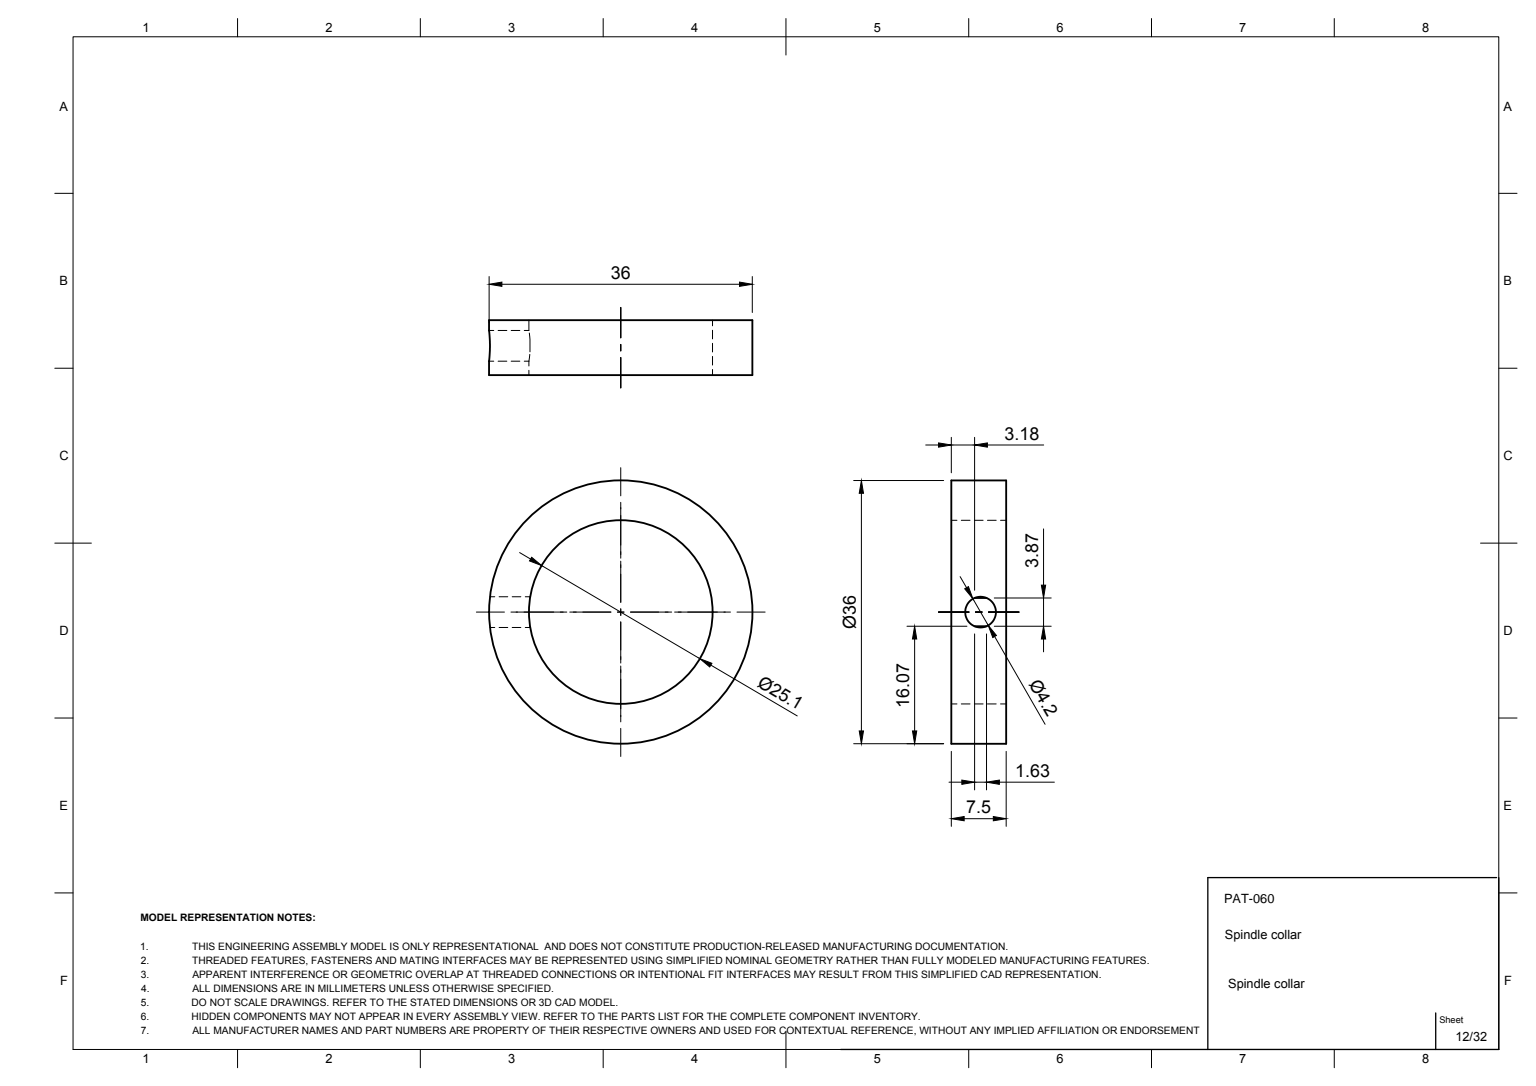
ISO-10303-21;
HEADER;
/* Generated by software containing ST-Developer
 * from STEP Tools, Inc. (www.steptools.com) 
 */

FILE_DESCRIPTION(
/* description */ ('Indexing fixture plate with plunger'),
/* implementation_level */ '2;1');

FILE_NAME(
/* name */ 'Spindle collar.step',
/* time_stamp */ '2026-10-28T03:23:41-07:00',
/* author */ (''),
/* organization */ (''),
/* preprocessor_version */ 'ST-DEVELOPER v20.2',
/* originating_system */ 'Autodesk Translation Framework v15.17.0.0',
/* authorisation */ '');

FILE_SCHEMA (('AUTOMOTIVE_DESIGN { 1 0 10303 214 3 1 1 }'));
ENDSEC;

DATA;
#10=MECHANICAL_DESIGN_GEOMETRIC_PRESENTATION_REPRESENTATION('',(#324),#10020);
#234=B_SPLINE_CURVE_WITH_KNOTS('',3,(#7309,#7310,#7311,#7312,#7313,#7314,
#7315,#7316,#7317,#7318,#7319,#7320,#7321,#7322),.UNSPECIFIED.,.F.,.F.,
(4,2,2,2,2,2,4),(0.714680326757343,0.792648662700719,0.871912238073926,
0.951175813447133,1.03043938882034,1.10970296419355,1.18767130013692),
 .UNSPECIFIED.);
#235=B_SPLINE_CURVE_WITH_KNOTS('',3,(#7326,#7327,#7328,#7329,#7330,#7331,
#7332,#7333),.UNSPECIFIED.,.F.,.F.,(4,2,2,4),(0.317058604482378,0.396322179855585,
0.475585755228792,0.55355409117217),.UNSPECIFIED.);
#236=B_SPLINE_CURVE_WITH_KNOTS('',3,(#7337,#7338,#7339,#7340,#7341,#7342,
#7343,#7344,#7345,#7346,#7347,#7348,#7349,#7350,#7351,#7352,#7353,#7354,
#7355,#7356,#7357,#7358,#7359,#7360,#7361,#7362),.UNSPECIFIED.,.F.,.F.,
(4,2,2,2,2,2,2,2,2,2,2,2,4),(0.,0.0791819055472369,0.158363811094474,0.237545215630596,
0.316726620166718,0.395908024702839,0.475089429238961,0.554271334786198,
0.633453240333435,0.712635145880672,0.791817051427909,0.870998455964031,
0.950179860500153),.UNSPECIFIED.);
#237=B_SPLINE_CURVE_WITH_KNOTS('',3,(#7363,#7364,#7365,#7366,#7367,#7368,
#7369,#7370,#7371,#7372),.UNSPECIFIED.,.F.,.F.,(4,2,2,2,4),(0.950179860500153,
1.02936126503627,1.1085426695724,1.18772457511963,1.26690648066687),
 .UNSPECIFIED.);
#238=B_SPLINE_CURVE_WITH_KNOTS('',3,(#7373,#7374,#7375,#7376,#7377,#7378,
#7379,#7380),.UNSPECIFIED.,.F.,.F.,(4,2,2,4),(0.0805631177925868,0.158531453735964,
0.237795029109171,0.317058604482378),.UNSPECIFIED.);
#270=SHAPE_REPRESENTATION_RELATIONSHIP('SRR','None',#10144,#297);
#297=ADVANCED_BREP_SHAPE_REPRESENTATION('',(#360),#9997);
#324=STYLED_ITEM('',(#10361),#360);
#360=MANIFOLD_SOLID_BREP('Body1',#4578);
#414=FACE_BOUND('',#1029,.T.);
#415=FACE_BOUND('',#1031,.T.);
#416=FACE_BOUND('',#1033,.T.);
#417=FACE_BOUND('',#1035,.T.);
#558=PLANE('',#5001);
#559=PLANE('',#5005);
#560=PLANE('',#5012);
#561=PLANE('',#5013);
#712=FACE_OUTER_BOUND('',#1025,.T.);
#713=FACE_OUTER_BOUND('',#1026,.T.);
#714=FACE_OUTER_BOUND('',#1027,.T.);
#715=FACE_OUTER_BOUND('',#1028,.T.);
#716=FACE_OUTER_BOUND('',#1030,.T.);
#717=FACE_OUTER_BOUND('',#1032,.T.);
#718=FACE_OUTER_BOUND('',#1034,.T.);
#1025=EDGE_LOOP('',(#3213,#3214));
#1026=EDGE_LOOP('',(#3215,#3216,#3217,#3218,#3219,#3220,#3221,#3222,#3223));
#1027=EDGE_LOOP('',(#3224,#3225));
#1028=EDGE_LOOP('',(#3226,#3227,#3228,#3229));
#1029=EDGE_LOOP('',(#3230,#3231,#3232,#3233,#3234));
#1030=EDGE_LOOP('',(#3235,#3236,#3237,#3238));
#1031=EDGE_LOOP('',(#3239,#3240));
#1032=EDGE_LOOP('',(#3241));
#1033=EDGE_LOOP('',(#3242));
#1034=EDGE_LOOP('',(#3243));
#1035=EDGE_LOOP('',(#3244));
#1425=LINE('',#7305,#1645);
#1426=LINE('',#7335,#1646);
#1427=LINE('',#7382,#1647);
#1428=LINE('',#7387,#1648);
#1429=LINE('',#7393,#1649);
#1645=VECTOR('',#5796,1.);
#1646=VECTOR('',#5803,0.21);
#1647=VECTOR('',#5806,1.);
#1648=VECTOR('',#5811,1.255);
#1649=VECTOR('',#5818,1.8);
#1874=CIRCLE('',#5002,0.21);
#1875=CIRCLE('',#5004,0.21);
#1876=CIRCLE('',#5007,1.255);
#1877=CIRCLE('',#5008,1.255);
#1878=CIRCLE('',#5010,1.8);
#1879=CIRCLE('',#5011,1.8);
#2185=VERTEX_POINT('',#7303);
#2186=VERTEX_POINT('',#7304);
#2187=VERTEX_POINT('',#7308);
#2188=VERTEX_POINT('',#7323);
#2189=VERTEX_POINT('',#7325);
#2190=VERTEX_POINT('',#7334);
#2191=VERTEX_POINT('',#7336);
#2192=VERTEX_POINT('',#7384);
#2193=VERTEX_POINT('',#7386);
#2194=VERTEX_POINT('',#7390);
#2195=VERTEX_POINT('',#7392);
#2586=EDGE_CURVE('',#2185,#2186,#1425,.T.);
#2587=EDGE_CURVE('',#2185,#2186,#1874,.T.);
#2588=EDGE_CURVE('',#2187,#2185,#234,.T.);
#2589=EDGE_CURVE('',#2188,#2187,#1875,.T.);
#2590=EDGE_CURVE('',#2189,#2188,#235,.T.);
#2591=EDGE_CURVE('',#2189,#2190,#1426,.T.);
#2592=EDGE_CURVE('',#2191,#2190,#236,.T.);
#2593=EDGE_CURVE('',#2190,#2191,#237,.T.);
#2594=EDGE_CURVE('',#2186,#2189,#238,.T.);
#2595=EDGE_CURVE('',#2188,#2187,#1427,.T.);
#2596=EDGE_CURVE('',#2192,#2192,#1876,.T.);
#2597=EDGE_CURVE('',#2192,#2193,#1428,.T.);
#2598=EDGE_CURVE('',#2193,#2193,#1877,.T.);
#2599=EDGE_CURVE('',#2194,#2194,#1878,.T.);
#2600=EDGE_CURVE('',#2194,#2195,#1429,.T.);
#2601=EDGE_CURVE('',#2195,#2195,#1879,.T.);
#3213=ORIENTED_EDGE('',*,*,#2586,.F.);
#3214=ORIENTED_EDGE('',*,*,#2587,.T.);
#3215=ORIENTED_EDGE('',*,*,#2588,.F.);
#3216=ORIENTED_EDGE('',*,*,#2589,.F.);
#3217=ORIENTED_EDGE('',*,*,#2590,.F.);
#3218=ORIENTED_EDGE('',*,*,#2591,.T.);
#3219=ORIENTED_EDGE('',*,*,#2592,.F.);
#3220=ORIENTED_EDGE('',*,*,#2593,.F.);
#3221=ORIENTED_EDGE('',*,*,#2591,.F.);
#3222=ORIENTED_EDGE('',*,*,#2594,.F.);
#3223=ORIENTED_EDGE('',*,*,#2587,.F.);
#3224=ORIENTED_EDGE('',*,*,#2595,.F.);
#3225=ORIENTED_EDGE('',*,*,#2589,.T.);
#3226=ORIENTED_EDGE('',*,*,#2596,.F.);
#3227=ORIENTED_EDGE('',*,*,#2597,.T.);
#3228=ORIENTED_EDGE('',*,*,#2598,.T.);
#3229=ORIENTED_EDGE('',*,*,#2597,.F.);
#3230=ORIENTED_EDGE('',*,*,#2594,.T.);
#3231=ORIENTED_EDGE('',*,*,#2590,.T.);
#3232=ORIENTED_EDGE('',*,*,#2595,.T.);
#3233=ORIENTED_EDGE('',*,*,#2588,.T.);
#3234=ORIENTED_EDGE('',*,*,#2586,.T.);
#3235=ORIENTED_EDGE('',*,*,#2599,.F.);
#3236=ORIENTED_EDGE('',*,*,#2600,.T.);
#3237=ORIENTED_EDGE('',*,*,#2601,.T.);
#3238=ORIENTED_EDGE('',*,*,#2600,.F.);
#3239=ORIENTED_EDGE('',*,*,#2592,.T.);
#3240=ORIENTED_EDGE('',*,*,#2593,.T.);
#3241=ORIENTED_EDGE('',*,*,#2599,.T.);
#3242=ORIENTED_EDGE('',*,*,#2596,.T.);
#3243=ORIENTED_EDGE('',*,*,#2601,.F.);
#3244=ORIENTED_EDGE('',*,*,#2598,.F.);
#4188=CYLINDRICAL_SURFACE('',#5003,0.21);
#4189=CYLINDRICAL_SURFACE('',#5006,1.255);
#4190=CYLINDRICAL_SURFACE('',#5009,1.8);
#4327=ADVANCED_FACE('',(#712),#558,.T.);
#4328=ADVANCED_FACE('',(#713),#4188,.F.);
#4329=ADVANCED_FACE('',(#714),#559,.T.);
#4330=ADVANCED_FACE('',(#715,#414),#4189,.F.);
#4331=ADVANCED_FACE('',(#716,#415),#4190,.T.);
#4332=ADVANCED_FACE('',(#717,#416),#560,.T.);
#4333=ADVANCED_FACE('',(#718,#417),#561,.F.);
#4578=CLOSED_SHELL('',(#4327,#4328,#4329,#4330,#4331,#4332,#4333));
#5000=AXIS2_PLACEMENT_3D('',#7301,#5792,#5793);
#5001=AXIS2_PLACEMENT_3D('',#7302,#5794,#5795);
#5002=AXIS2_PLACEMENT_3D('',#7306,#5797,#5798);
#5003=AXIS2_PLACEMENT_3D('',#7307,#5799,#5800);
#5004=AXIS2_PLACEMENT_3D('',#7324,#5801,#5802);
#5005=AXIS2_PLACEMENT_3D('',#7381,#5804,#5805);
#5006=AXIS2_PLACEMENT_3D('',#7383,#5807,#5808);
#5007=AXIS2_PLACEMENT_3D('',#7385,#5809,#5810);
#5008=AXIS2_PLACEMENT_3D('',#7388,#5812,#5813);
#5009=AXIS2_PLACEMENT_3D('',#7389,#5814,#5815);
#5010=AXIS2_PLACEMENT_3D('',#7391,#5816,#5817);
#5011=AXIS2_PLACEMENT_3D('',#7394,#5819,#5820);
#5012=AXIS2_PLACEMENT_3D('',#7395,#5821,#5822);
#5013=AXIS2_PLACEMENT_3D('',#7396,#5823,#5824);
#5792=DIRECTION('axis',(0.,0.,1.));
#5793=DIRECTION('refdir',(1.,0.,0.));
#5794=DIRECTION('center_axis',(1.,0.,0.));
#5795=DIRECTION('ref_axis',(0.,0.,-1.));
#5796=DIRECTION('',(0.,0.,1.));
#5797=DIRECTION('center_axis',(1.,0.,0.));
#5798=DIRECTION('ref_axis',(0.,0.,-1.));
#5799=DIRECTION('center_axis',(1.,0.,0.));
#5800=DIRECTION('ref_axis',(0.,0.,-1.));
#5801=DIRECTION('center_axis',(1.,0.,0.));
#5802=DIRECTION('ref_axis',(0.,0.,-1.));
#5803=DIRECTION('',(1.,0.,0.));
#5804=DIRECTION('center_axis',(1.,0.,0.));
#5805=DIRECTION('ref_axis',(0.,0.,-1.));
#5806=DIRECTION('',(0.,0.,-1.));
#5807=DIRECTION('center_axis',(0.,0.,1.));
#5808=DIRECTION('ref_axis',(1.,0.,0.));
#5809=DIRECTION('center_axis',(0.,0.,-1.));
#5810=DIRECTION('ref_axis',(1.,0.,0.));
#5811=DIRECTION('',(0.,0.,-1.));
#5812=DIRECTION('center_axis',(0.,0.,-1.));
#5813=DIRECTION('ref_axis',(1.,0.,0.));
#5814=DIRECTION('center_axis',(0.,0.,1.));
#5815=DIRECTION('ref_axis',(1.,0.,0.));
#5816=DIRECTION('center_axis',(0.,0.,1.));
#5817=DIRECTION('ref_axis',(1.,0.,0.));
#5818=DIRECTION('',(0.,0.,-1.));
#5819=DIRECTION('center_axis',(0.,0.,1.));
#5820=DIRECTION('ref_axis',(1.,0.,0.));
#5821=DIRECTION('center_axis',(0.,0.,1.));
#5822=DIRECTION('ref_axis',(1.,0.,0.));
#5823=DIRECTION('center_axis',(0.,0.,1.));
#5824=DIRECTION('ref_axis',(1.,0.,0.));
#7301=CARTESIAN_POINT('',(0.,0.,0.));
#7302=CARTESIAN_POINT('Origin',(1.24,0.,6.6));
#7303=CARTESIAN_POINT('',(1.24,0.19345542122153,6.51829932680816));
#7304=CARTESIAN_POINT('',(1.24,0.19345542122153,6.68170067319184));
#7305=CARTESIAN_POINT('',(1.24,0.193455421221531,6.25));
#7306=CARTESIAN_POINT('Origin',(1.24,0.,6.6));
#7307=CARTESIAN_POINT('Origin',(1.24,0.,6.6));
#7308=CARTESIAN_POINT('',(1.24,-0.19345542122153,6.51829932680816));
#7309=CARTESIAN_POINT('Ctrl Pts',(1.24,-0.193455421221531,6.51829932680816));
#7310=CARTESIAN_POINT('Ctrl Pts',(1.24167145707784,-0.182741806873435,6.49293103184137));
#7311=CARTESIAN_POINT('Ctrl Pts',(1.24400210952839,-0.16680484953796,6.46982000143961));
#7312=CARTESIAN_POINT('Ctrl Pts',(1.24840249136865,-0.129875785635207,6.43289093753686));
#7313=CARTESIAN_POINT('Ctrl Pts',(1.2507589672592,-0.106295060941802,6.4167372734261));
#7314=CARTESIAN_POINT('Ctrl Pts',(1.25408084670822,-0.0545698089447939,
6.39529044194989));
#7315=CARTESIAN_POINT('Ctrl Pts',(1.255,-0.0264211917910691,6.39));
#7316=CARTESIAN_POINT('Ctrl Pts',(1.255,0.026421191791069,6.39));
#7317=CARTESIAN_POINT('Ctrl Pts',(1.25408084670822,0.0545698089447938,6.39529044194989));
#7318=CARTESIAN_POINT('Ctrl Pts',(1.2507589672592,0.106295060941802,6.4167372734261));
#7319=CARTESIAN_POINT('Ctrl Pts',(1.24840249136865,0.129875785635207,6.43289093753686));
#7320=CARTESIAN_POINT('Ctrl Pts',(1.24400210952839,0.166804849537961,6.46982000143961));
#7321=CARTESIAN_POINT('Ctrl Pts',(1.24167145707784,0.182741806873435,6.49293103184137));
#7322=CARTESIAN_POINT('Ctrl Pts',(1.24,0.193455421221531,6.51829932680816));
#7323=CARTESIAN_POINT('',(1.24,-0.19345542122153,6.68170067319184));
#7324=CARTESIAN_POINT('Origin',(1.24,0.,6.6));
#7325=CARTESIAN_POINT('',(1.255,-5.44921548144906E-17,6.81));
#7326=CARTESIAN_POINT('Ctrl Pts',(1.255,-3.46944695195361E-17,6.81));
#7327=CARTESIAN_POINT('Ctrl Pts',(1.255,-0.0264211917910691,6.81));
#7328=CARTESIAN_POINT('Ctrl Pts',(1.25408084670822,-0.0545698089447938,
6.80470955805011));
#7329=CARTESIAN_POINT('Ctrl Pts',(1.2507589672592,-0.106295060941802,6.7832627265739));
#7330=CARTESIAN_POINT('Ctrl Pts',(1.24840249136865,-0.129875785635207,6.76710906246314));
#7331=CARTESIAN_POINT('Ctrl Pts',(1.24400210952839,-0.166804849537961,6.73017999856039));
#7332=CARTESIAN_POINT('Ctrl Pts',(1.24167145707784,-0.182741806873434,6.70706896815863));
#7333=CARTESIAN_POINT('Ctrl Pts',(1.24,-0.193455421221531,6.68170067319184));
#7334=CARTESIAN_POINT('',(1.8,-2.57175827820944E-17,6.81));
#7335=CARTESIAN_POINT('',(1.24,-2.57175827820944E-17,6.81));
#7336=CARTESIAN_POINT('',(1.78770802985275,0.21,6.6));
#7337=CARTESIAN_POINT('Ctrl Pts',(1.78770802985275,0.21,6.6));
#7338=CARTESIAN_POINT('Ctrl Pts',(1.78770802985275,0.21,6.57360603148425));
#7339=CARTESIAN_POINT('Ctrl Pts',(1.78835284034214,0.204720232951726,6.54546934556601));
#7340=CARTESIAN_POINT('Ctrl Pts',(1.79067700538683,0.1832815239789,6.49373688397397));
#7341=CARTESIAN_POINT('Ctrl Pts',(1.79232226897314,0.167123888882363,6.47013904078401));
#7342=CARTESIAN_POINT('Ctrl Pts',(1.79540680803063,0.129861077103665,6.43287622900531));
#7343=CARTESIAN_POINT('Ctrl Pts',(1.79704717240673,0.106263182528071,6.4167185016358));
#7344=CARTESIAN_POINT('Ctrl Pts',(1.79936011492601,0.0545305475112077,6.39527972468261));
#7345=CARTESIAN_POINT('Ctrl Pts',(1.8,0.0263938015120406,6.39));
#7346=CARTESIAN_POINT('Ctrl Pts',(1.8,-0.0263938015120406,6.39));
#7347=CARTESIAN_POINT('Ctrl Pts',(1.79936011492601,-0.0545305475112077,
6.39527972468261));
#7348=CARTESIAN_POINT('Ctrl Pts',(1.79704717240673,-0.106263182528071,6.4167185016358));
#7349=CARTESIAN_POINT('Ctrl Pts',(1.79540680803063,-0.129861077103665,6.43287622900531));
#7350=CARTESIAN_POINT('Ctrl Pts',(1.79232226897314,-0.167123888882363,6.47013904078401));
#7351=CARTESIAN_POINT('Ctrl Pts',(1.79067700538683,-0.1832815239789,6.49373688397397));
#7352=CARTESIAN_POINT('Ctrl Pts',(1.78835284034214,-0.204720232951726,6.54546934556602));
#7353=CARTESIAN_POINT('Ctrl Pts',(1.78770802985275,-0.21,6.57360603148425));
#7354=CARTESIAN_POINT('Ctrl Pts',(1.78770802985275,-0.21,6.62639396851575));
#7355=CARTESIAN_POINT('Ctrl Pts',(1.78835284034214,-0.204720232951726,6.65453065443398));
#7356=CARTESIAN_POINT('Ctrl Pts',(1.79067700538683,-0.1832815239789,6.70626311602603));
#7357=CARTESIAN_POINT('Ctrl Pts',(1.79232226897314,-0.167123888882363,6.72986095921599));
#7358=CARTESIAN_POINT('Ctrl Pts',(1.79540680803063,-0.129861077103665,6.76712377099468));
#7359=CARTESIAN_POINT('Ctrl Pts',(1.79704717240673,-0.106263182528071,6.7832814983642));
#7360=CARTESIAN_POINT('Ctrl Pts',(1.79936011492601,-0.0545305475112076,
6.80472027531739));
#7361=CARTESIAN_POINT('Ctrl Pts',(1.8,-0.0263938015120407,6.81));
#7362=CARTESIAN_POINT('Ctrl Pts',(1.8,-6.93889390390723E-17,6.81));
#7363=CARTESIAN_POINT('Ctrl Pts',(1.8,-2.77555756156289E-17,6.81));
#7364=CARTESIAN_POINT('Ctrl Pts',(1.8,0.0263938015120406,6.81));
#7365=CARTESIAN_POINT('Ctrl Pts',(1.79936011492601,0.0545305475112076,6.80472027531739));
#7366=CARTESIAN_POINT('Ctrl Pts',(1.79704717240673,0.106263182528071,6.7832814983642));
#7367=CARTESIAN_POINT('Ctrl Pts',(1.79540680803063,0.129861077103665,6.76712377099468));
#7368=CARTESIAN_POINT('Ctrl Pts',(1.79232226897314,0.167123888882363,6.72986095921599));
#7369=CARTESIAN_POINT('Ctrl Pts',(1.79067700538683,0.1832815239789,6.70626311602603));
#7370=CARTESIAN_POINT('Ctrl Pts',(1.78835284034214,0.204720232951726,6.65453065443398));
#7371=CARTESIAN_POINT('Ctrl Pts',(1.78770802985275,0.21,6.62639396851575));
#7372=CARTESIAN_POINT('Ctrl Pts',(1.78770802985275,0.21,6.6));
#7373=CARTESIAN_POINT('Ctrl Pts',(1.24,0.193455421221531,6.68170067319184));
#7374=CARTESIAN_POINT('Ctrl Pts',(1.24167145707784,0.182741806873435,6.70706896815863));
#7375=CARTESIAN_POINT('Ctrl Pts',(1.24400210952839,0.166804849537961,6.73017999856039));
#7376=CARTESIAN_POINT('Ctrl Pts',(1.24840249136865,0.129875785635207,6.76710906246314));
#7377=CARTESIAN_POINT('Ctrl Pts',(1.2507589672592,0.106295060941802,6.7832627265739));
#7378=CARTESIAN_POINT('Ctrl Pts',(1.25408084670822,0.0545698089447938,6.80470955805011));
#7379=CARTESIAN_POINT('Ctrl Pts',(1.255,0.0264211917910689,6.81));
#7380=CARTESIAN_POINT('Ctrl Pts',(1.255,-8.32667268468867E-17,6.81));
#7381=CARTESIAN_POINT('Origin',(1.24,0.,6.6));
#7382=CARTESIAN_POINT('',(1.24,-0.193455421221531,6.25));
#7383=CARTESIAN_POINT('Origin',(0.,0.,6.25));
#7384=CARTESIAN_POINT('',(-1.255,-1.53693173292993E-16,7.));
#7385=CARTESIAN_POINT('Origin',(0.,0.,7.));
#7386=CARTESIAN_POINT('',(-1.255,-1.53693173292993E-16,6.25));
#7387=CARTESIAN_POINT('',(-1.255,-1.53693173292993E-16,6.25));
#7388=CARTESIAN_POINT('Origin',(0.,0.,6.25));
#7389=CARTESIAN_POINT('Origin',(0.,0.,6.25));
#7390=CARTESIAN_POINT('',(-1.8,-2.20436423846524E-16,7.));
#7391=CARTESIAN_POINT('Origin',(0.,0.,7.));
#7392=CARTESIAN_POINT('',(-1.8,-2.20436423846524E-16,6.25));
#7393=CARTESIAN_POINT('',(-1.8,-2.20436423846524E-16,6.25));
#7394=CARTESIAN_POINT('Origin',(0.,0.,6.25));
#7395=CARTESIAN_POINT('Origin',(0.,0.,7.));
#7396=CARTESIAN_POINT('Origin',(0.,0.,6.25));
#9964=UNCERTAINTY_MEASURE_WITH_UNIT(LENGTH_MEASURE(0.001),#10021,
'DISTANCE_ACCURACY_VALUE',
'Maximum model space distance between geometric entities at asserted c
onnectivities');
#9987=UNCERTAINTY_MEASURE_WITH_UNIT(LENGTH_MEASURE(0.001),#10021,
'DISTANCE_ACCURACY_VALUE',
'Maximum model space distance between geometric entities at asserted c
onnectivities');
#9997=(
GEOMETRIC_REPRESENTATION_CONTEXT(3)
GLOBAL_UNCERTAINTY_ASSIGNED_CONTEXT((#9964))
GLOBAL_UNIT_ASSIGNED_CONTEXT((#10021,#10023,#10024))
REPRESENTATION_CONTEXT('','3D')
);
#10020=(
GEOMETRIC_REPRESENTATION_CONTEXT(3)
GLOBAL_UNCERTAINTY_ASSIGNED_CONTEXT((#9987))
GLOBAL_UNIT_ASSIGNED_CONTEXT((#10021,#10023,#10024))
REPRESENTATION_CONTEXT('','3D')
);
#10021=(
LENGTH_UNIT()
NAMED_UNIT(*)
SI_UNIT(.CENTI.,.METRE.)
);
#10023=(
NAMED_UNIT(*)
PLANE_ANGLE_UNIT()
SI_UNIT($,.RADIAN.)
);
#10024=(
NAMED_UNIT(*)
SI_UNIT($,.STERADIAN.)
SOLID_ANGLE_UNIT()
);
#10034=SHAPE_DEFINITION_REPRESENTATION(#10066,#10144);
#10066=PRODUCT_DEFINITION_SHAPE('',$,#10177);
#10144=SHAPE_REPRESENTATION('',(#5000),#9997);
#10167=PRODUCT_DEFINITION_CONTEXT('part definition',#10265,'design');
#10177=PRODUCT_DEFINITION('Spindle collar','Spindle collar',#10209,#10167);
#10209=PRODUCT_DEFINITION_FORMATION('',$,#10276);
#10265=APPLICATION_CONTEXT(
'Core Data for Automotive Mechanical Design Process');
#10266=PRODUCT_CONTEXT('part definition',#10265,'mechanical');
#10276=PRODUCT('Spindle collar','Spindle collar','Spindle collar',(#10266));
#10355=COLOUR_RGB('Sky Blue',0.24,0.69,0.87);
#10356=FILL_AREA_STYLE_COLOUR('',#10355);
#10357=FILL_AREA_STYLE('',(#10356));
#10358=SURFACE_STYLE_FILL_AREA(#10357);
#10359=SURFACE_SIDE_STYLE('',(#10358));
#10360=SURFACE_STYLE_USAGE(.BOTH.,#10359);
#10361=PRESENTATION_STYLE_ASSIGNMENT((#10360));
ENDSEC;
END-ISO-10303-21;
